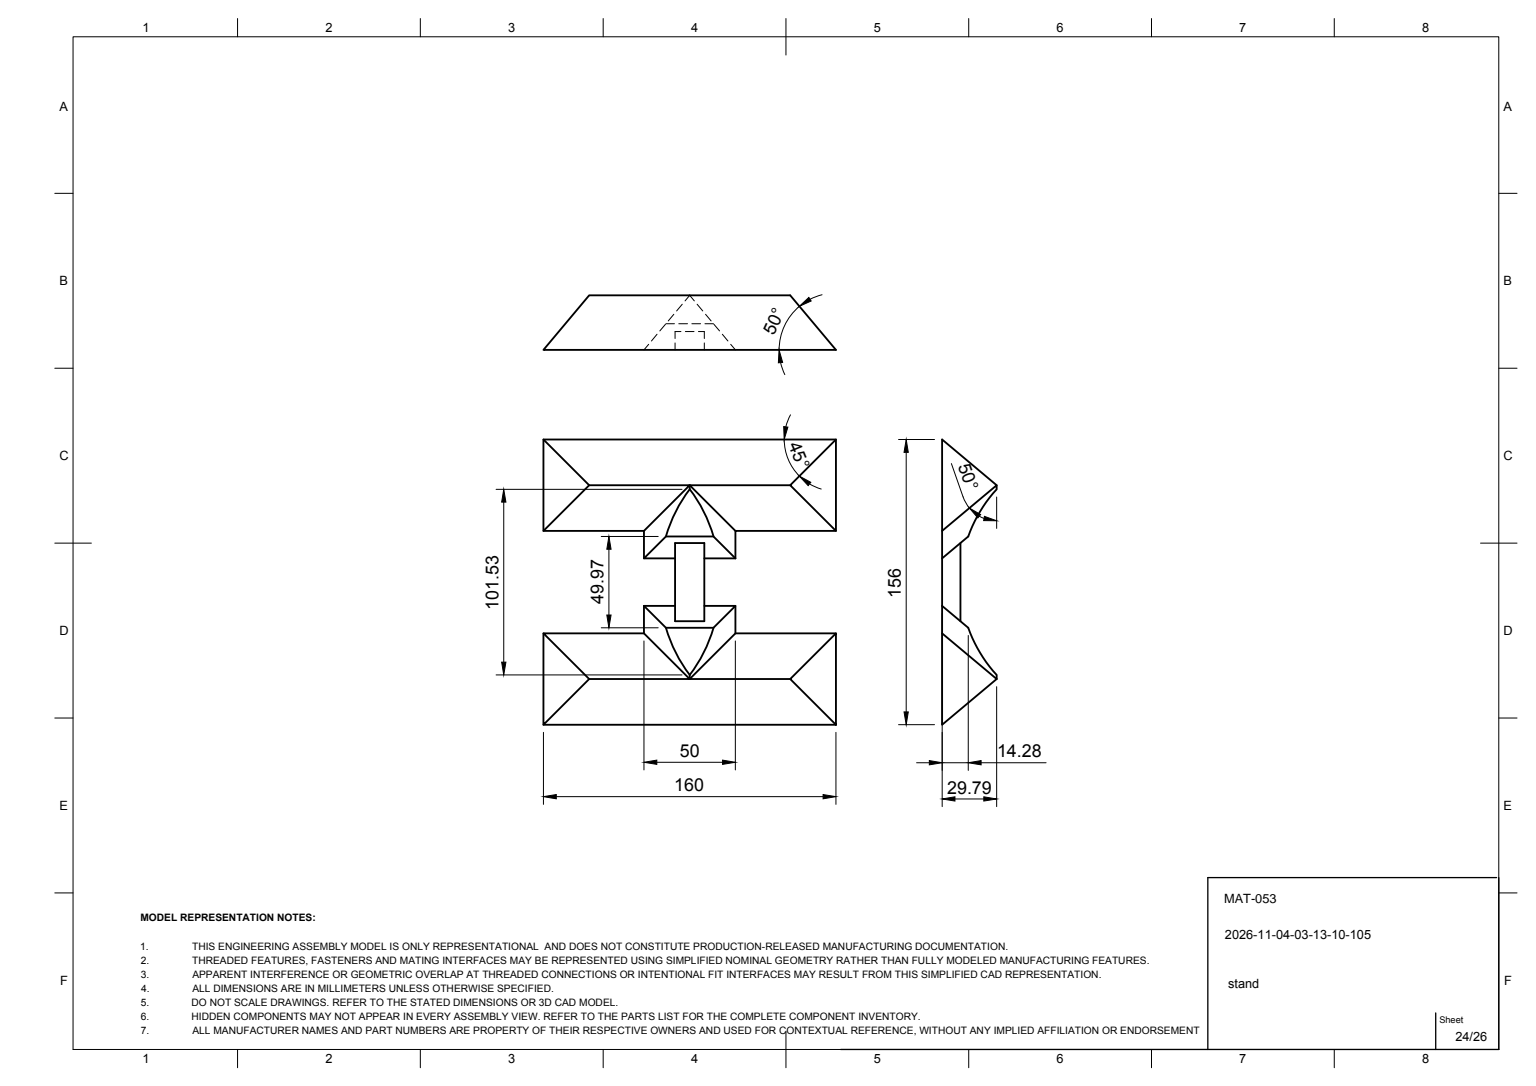
ISO-10303-21;
HEADER;
FILE_DESCRIPTION (('STEP AP214'),
    '1' );
FILE_NAME ('stand.step',
    '2026-10-10T03:43:58',
    ( '' ),
    ( '' ),
    'SwSTEP 2.0',
    'SolidWorks 2026',
    '' );
FILE_SCHEMA (( 'AUTOMOTIVE_DESIGN' ));
ENDSEC;

DATA;
#146=EDGE_LOOP ( 'NONE', ( #8104, #20994, #5292, #47649 ) ) ;
#193=( BOUNDED_CURVE ( )  B_SPLINE_CURVE ( 3, ( #51309, #3119, #36157, #51647 ),
 .UNSPECIFIED., .F., .F. ) 
 B_SPLINE_CURVE_WITH_KNOTS ( ( 4, 4 ),
 ( 0.3396391817068888930, 0.7435323497954801075 ),
 .UNSPECIFIED. ) 
 CURVE ( )  GEOMETRIC_REPRESENTATION_ITEM ( )  RATIONAL_B_SPLINE_CURVE ( ( 1.000000000000000000, 0.9864519964717846090, 0.9864519964717846090, 1.000000000000000000 ) ) 
 REPRESENTATION_ITEM ( '' )  );
#273=CARTESIAN_POINT ( 'NONE',  ( -34.39099631177280969, 10.00000000000000000, -33.00000000000000000 ) ) ;
#625=( BOUNDED_CURVE ( )  B_SPLINE_CURVE ( 3, ( #39954, #62719, #29065, #46526 ),
 .UNSPECIFIED., .F., .F. ) 
 B_SPLINE_CURVE_WITH_KNOTS ( ( 4, 4 ),
 ( 3.481231835296680899, 3.885125003385272446 ),
 .UNSPECIFIED. ) 
 CURVE ( )  GEOMETRIC_REPRESENTATION_ITEM ( )  RATIONAL_B_SPLINE_CURVE ( ( 1.000000000000000000, 0.9864519964717846090, 0.9864519964717846090, 1.000000000000000000 ) ) 
 REPRESENTATION_ITEM ( '' )  );
#713=AXIS2_PLACEMENT_3D ( 'NONE', #6914, #44550, #24147 ) ;
#793=DIRECTION ( 'NONE',  ( -1.661094098900087138E-16, 0.6427876096865404731, 0.7660444431189771253 ) ) ;
#1281=CARTESIAN_POINT ( 'NONE',  ( -26.00000000000000000, 0.000000000000000000, -2.818925648462311923E-15 ) ) ;
#1484=DIRECTION ( 'NONE',  ( 0.000000000000000000, -1.000000000000000000, 0.000000000000000000 ) ) ;
#1494=ADVANCED_FACE ( 'NONE', ( #31724 ), #63402, .T. ) ;
#1497=LINE ( 'NONE', #6064, #10599 ) ;
#1562=DIRECTION ( 'NONE',  ( -1.393823445737823288E-16, 0.7660444431189770143, 0.6427876096865403621 ) ) ;
#1581=VECTOR ( 'NONE', #15769, 1000.000000000000000 ) ;
#1761=EDGE_CURVE ( 'NONE', #54242, #40885, #49448, .T. ) ;
#1806=LINE ( 'NONE', #55245, #35511 ) ;
#1841=CARTESIAN_POINT ( 'NONE',  ( -12.99999999999999645, 0.000000000000000000, -33.00000000000000000 ) ) ;
#1965=CARTESIAN_POINT ( 'NONE',  ( 45.69927128652683734, 36.58596684574255420, -74.30072871347310581 ) ) ;
#2144=LINE ( 'NONE', #35537, #4043 ) ;
#2191=ORIENTED_EDGE ( 'NONE', *, *, #45440, .F. ) ;
#2230=ORIENTED_EDGE ( 'NONE', *, *, #34718, .T. ) ;
#2285=DIRECTION ( 'NONE',  ( 0.5407162030609372616, -0.6444004775717706579, -0.5407162030609374836 ) ) ;
#2317=CARTESIAN_POINT ( 'NONE',  ( 14.99999999999997158, 0.000000000000000000, -0.000000000000000000 ) ) ;
#2392=VERTEX_POINT ( 'NONE', #7790 ) ;
#2515=LINE ( 'NONE', #29246, #19698 ) ;
#2527=ADVANCED_FACE ( 'NONE', ( #21112 ), #68930, .T. ) ;
#2596=DIRECTION ( 'NONE',  ( -2.168404344971009361E-16, 0.000000000000000000, 1.000000000000000000 ) ) ;
#2611=PLANE ( 'NONE',  #12739 ) ;
#2686=FACE_OUTER_BOUND ( 'NONE', #48013, .T. ) ;
#2724=ORIENTED_EDGE ( 'NONE', *, *, #21371, .T. ) ;
#2912=VERTEX_POINT ( 'NONE', #20576 ) ;
#3017=ORIENTED_EDGE ( 'NONE', *, *, #44711, .T. ) ;
#3061=ORIENTED_EDGE ( 'NONE', *, *, #6840, .F. ) ;
#3119=CARTESIAN_POINT ( 'NONE',  ( 21.57182537987934978, 17.67134260003773960, -35.17198294190094288 ) ) ;
#3171=EDGE_LOOP ( 'NONE', ( #50531, #3061, #20090 ) ) ;
#3185=DIRECTION ( 'NONE',  ( -2.168404344971009361E-16, 0.000000000000000000, 1.000000000000000000 ) ) ;
#3231=CARTESIAN_POINT ( 'NONE',  ( 14.99999999999997158, 0.000000000000000000, -50.00000000000000000 ) ) ;
#3532=APPLICATION_CONTEXT ( 'automotive_design' ) ;
#3575=EDGE_LOOP ( 'NONE', ( #20280, #65714, #25182, #9840, #14109 ) ) ;
#3588=PRODUCT_DEFINITION_SHAPE ( 'NONE', 'NONE',  #45241 ) ;
#3605=DIRECTION ( 'NONE',  ( -0.000000000000000000, -0.000000000000000000, 1.000000000000000000 ) ) ;
#3821=ADVANCED_FACE ( 'NONE', ( #39549 ), #2611, .T. ) ;
#3956=LINE ( 'NONE', #25073, #49414 ) ;
#3992=CARTESIAN_POINT ( 'NONE',  ( 0.000000000000000000, 0.000000000000000000, -50.00000000000000000 ) ) ;
#4002=LINE ( 'NONE', #9970, #39539 ) ;
#4043=VECTOR ( 'NONE', #45035, 1000.000000000000000 ) ;
#4119=LINE ( 'NONE', #41409, #61177 ) ;
#4213=DIRECTION ( 'NONE',  ( 1.000000000000000000, -0.000000000000000000, 0.000000000000000000 ) ) ;
#4408=LINE ( 'NONE', #25872, #23224 ) ;
#4594=ADVANCED_FACE ( 'NONE', ( #49482 ), #33688, .F. ) ;
#4687=CARTESIAN_POINT ( 'NONE',  ( 8.390996311772815019, 10.00000000000000000, -33.00000000000000000 ) ) ;
#4737=EDGE_LOOP ( 'NONE', ( #2724, #13378, #43528, #13191 ) ) ;
#4784=DIRECTION ( 'NONE',  ( 8.673617379884039170E-17, 1.033681467326434846E-16, 1.000000000000000000 ) ) ;
#4834=VECTOR ( 'NONE', #51632, 1000.000000000000000 ) ;
#4901=DIRECTION ( 'NONE',  ( 0.6427876096865403621, -0.7660444431189770143, 1.393823445737823288E-16 ) ) ;
#4994=VERTEX_POINT ( 'NONE', #18285 ) ;
#5189=ORIENTED_EDGE ( 'NONE', *, *, #28493, .T. ) ;
#5193=EDGE_CURVE ( 'NONE', #30932, #4994, #40774, .T. ) ;
#5249=FACE_OUTER_BOUND ( 'NONE', #17680, .T. ) ;
#5292=ORIENTED_EDGE ( 'NONE', *, *, #45012, .T. ) ;
#5325=EDGE_CURVE ( 'NONE', #62792, #66752, #31273, .T. ) ;
#5335=DIRECTION ( 'NONE',  ( -0.7660444431189771253, 0.6427876096865404731, 0.000000000000000000 ) ) ;
#5465=VERTEX_POINT ( 'NONE', #273 ) ;
#5614=EDGE_LOOP ( 'NONE', ( #66785, #60378, #47106, #7908 ) ) ;
#5643=CARTESIAN_POINT ( 'NONE',  ( 37.76691715686636996, 29.79383981485516841, -24.99999999999999645 ) ) ;
#5828=PLANE ( 'NONE',  #42178 ) ;
#5906=EDGE_CURVE ( 'NONE', #52737, #43093, #57568, .T. ) ;
#6064=CARTESIAN_POINT ( 'NONE',  ( 11.98601804829806383, 14.28438006995820508, 82.99999999999998579 ) ) ;
#6095=ADVANCED_FACE ( 'NONE', ( #31440 ), #33082, .T. ) ;
#6395=ORIENTED_EDGE ( 'NONE', *, *, #53817, .T. ) ;
#6399=AXIS2_PLACEMENT_3D ( 'NONE', #58013, #42520, #46760 ) ;
#6403=ORIENTED_EDGE ( 'NONE', *, *, #61855, .T. ) ;
#6489=ORIENTED_EDGE ( 'NONE', *, *, #62229, .T. ) ;
#6521=CARTESIAN_POINT ( 'NONE',  ( -37.98601804829807094, 14.28438006995821219, -38.01398195170192906 ) ) ;
#6640=FILL_AREA_STYLE_COLOUR ( '', #26224 ) ;
#6752=LINE ( 'NONE', #54222, #44139 ) ;
#6808=EDGE_CURVE ( 'NONE', #52737, #49963, #59288, .T. ) ;
#6840=EDGE_CURVE ( 'NONE', #10412, #60955, #55768, .T. ) ;
#6914=CARTESIAN_POINT ( 'NONE',  ( -25.99999999999994671, 0.000000000000000000, -104.9999999999999858 ) ) ;
#7029=ORIENTED_EDGE ( 'NONE', *, *, #45012, .F. ) ;
#7036=EDGE_LOOP ( 'NONE', ( #18856, #65533, #68042 ) ) ;
#7077=ORIENTED_EDGE ( 'NONE', *, *, #12957, .F. ) ;
#7275=PLANE ( 'NONE',  #36813 ) ;
#7545=DIRECTION ( 'NONE',  ( -1.000000000000000000, 0.000000000000000000, -0.000000000000000000 ) ) ;
#7708=VERTEX_POINT ( 'NONE', #8980 ) ;
#7790=CARTESIAN_POINT ( 'NONE',  ( -25.99999999999998934, 0.000000000000000000, -50.00000000000000000 ) ) ;
#7908=ORIENTED_EDGE ( 'NONE', *, *, #5906, .F. ) ;
#7927=ORIENTED_EDGE ( 'NONE', *, *, #36685, .T. ) ;
#7960=FACE_OUTER_BOUND ( 'NONE', #31655, .T. ) ;
#8104=ORIENTED_EDGE ( 'NONE', *, *, #5325, .F. ) ;
#8310=CARTESIAN_POINT ( 'NONE',  ( 48.91942932610495376, 19.16407787157945108, 38.91942932610497508 ) ) ;
#8319=DIRECTION ( 'NONE',  ( 1.000000000000000000, 0.000000000000000000, 0.000000000000000000 ) ) ;
#8444=CYLINDRICAL_SURFACE ( 'NONE', #53975, 75.00000000000001421 ) ;
#8520=VERTEX_POINT ( 'NONE', #36152 ) ;
#8591=EDGE_CURVE ( 'NONE', #52737, #53508, #16066, .T. ) ;
#8980=CARTESIAN_POINT ( 'NONE',  ( 11.98601804829806561, 14.28438006995821219, -38.01398195170192906 ) ) ;
#9083=LINE ( 'NONE', #68181, #56913 ) ;
#9198=CARTESIAN_POINT ( 'NONE',  ( -25.99999999999998934, 0.000000000000000000, -50.00000000000000000 ) ) ;
#9199=CARTESIAN_POINT ( 'NONE',  ( -40.99999999999994316, 0.000000000000000000, -104.9999999999999858 ) ) ;
#9378=CARTESIAN_POINT ( 'NONE',  ( -65.99999999999997158, 29.79383981485517197, -2.367957528293540247E-14 ) ) ;
#9391=ADVANCED_FACE ( 'NONE', ( #10501 ), #15452, .T. ) ;
#9660=CARTESIAN_POINT ( 'NONE',  ( -36.61438981621041933, -5.226566692248928447, -54.38561018378954515 ) ) ;
#9758=LINE ( 'NONE', #15026, #4834 ) ;
#9840=ORIENTED_EDGE ( 'NONE', *, *, #30834, .F. ) ;
#9859=VECTOR ( 'NONE', #53368, 1000.000000000000000 ) ;
#9970=CARTESIAN_POINT ( 'NONE',  ( 0.000000000000000000, 0.000000000000000000, -33.00000000000000000 ) ) ;
#9978=CARTESIAN_POINT ( 'NONE',  ( 0.000000000000000000, 0.000000000000000000, -33.00000000000000000 ) ) ;
#10324=CARTESIAN_POINT ( 'NONE',  ( -3.469446951953614189E-15, 0.000000000000000000, -17.00000000000000355 ) ) ;
#10345=EDGE_LOOP ( 'NONE', ( #24574, #33856, #6403 ) ) ;
#10412=VERTEX_POINT ( 'NONE', #57416 ) ;
#10439=ORIENTED_EDGE ( 'NONE', *, *, #58459, .T. ) ;
#10501=FACE_OUTER_BOUND ( 'NONE', #5614, .T. ) ;
#10587=VECTOR ( 'NONE', #12206, 1000.000000000000114 ) ;
#10599=VECTOR ( 'NONE', #44406, 1000.000000000000000 ) ;
#10755=ORIENTED_EDGE ( 'NONE', *, *, #61855, .F. ) ;
#10830=DIRECTION ( 'NONE',  ( 0.000000000000000000, 0.000000000000000000, -1.000000000000000000 ) ) ;
#10864=CARTESIAN_POINT ( 'NONE',  ( -26.00000000000000000, 0.000000000000000000, -2.818925648462311923E-15 ) ) ;
#10931=DIRECTION ( 'NONE',  ( -2.724194322196142817E-16, 0.6427876096865404731, 0.7660444431189771253 ) ) ;
#11112=FACE_OUTER_BOUND ( 'NONE', #3171, .T. ) ;
#11205=LINE ( 'NONE', #31985, #66301 ) ;
#11331=CARTESIAN_POINT ( 'NONE',  ( -37.98601804829808515, 14.28438006995824772, -11.98601804829809581 ) ) ;
#11336=LINE ( 'NONE', #54236, #62534 ) ;
#11370=CARTESIAN_POINT ( 'NONE',  ( -12.99999999999999822, 10.00000000000000000, -17.00000000000000355 ) ) ;
#11437=CARTESIAN_POINT ( 'NONE',  ( -65.99999999999998579, 29.79383981485516841, -1.674068137902818041E-14 ) ) ;
#11515=LINE ( 'NONE', #9198, #39329 ) ;
#11760=CARTESIAN_POINT ( 'NONE',  ( -25.99999999999998934, 0.000000000000000000, -50.00000000000000000 ) ) ;
#11826=DIRECTION ( 'NONE',  ( 0.5407162030609375947, -0.6444004775717707689, -0.5407162030609372616 ) ) ;
#12206=DIRECTION ( 'NONE',  ( -0.6427876096865403621, 0.7660444431189770143, -5.360859406683936151E-17 ) ) ;
#12293=ORIENTED_EDGE ( 'NONE', *, *, #16445, .T. ) ;
#12294=ORIENTED_EDGE ( 'NONE', *, *, #61559, .T. ) ;
#12424=CARTESIAN_POINT ( 'NONE',  ( 7.632783294297949638E-15, 0.000000000000000000, 55.00000000000001421 ) ) ;
#12567=ORIENTED_EDGE ( 'NONE', *, *, #34694, .T. ) ;
#12724=VECTOR ( 'NONE', #21195, 1000.000000000000114 ) ;
#12739=AXIS2_PLACEMENT_3D ( 'NONE', #11760, #33932, #1562 ) ;
#12957=EDGE_CURVE ( 'NONE', #34803, #30932, #56987, .T. ) ;
#12975=ORIENTED_EDGE ( 'NONE', *, *, #17452, .F. ) ;
#13191=ORIENTED_EDGE ( 'NONE', *, *, #47317, .F. ) ;
#13222=VECTOR ( 'NONE', #28910, 1000.000000000000114 ) ;
#13378=ORIENTED_EDGE ( 'NONE', *, *, #37390, .T. ) ;
#13701=CARTESIAN_POINT ( 'NONE',  ( 14.99999999999998579, 0.000000000000000000, -0.000000000000000000 ) ) ;
#13768=EDGE_CURVE ( 'NONE', #40885, #66752, #11205, .T. ) ;
#13823=EDGE_CURVE ( 'NONE', #41104, #30932, #38646, .T. ) ;
#14076=EDGE_CURVE ( 'NONE', #43093, #19218, #48063, .T. ) ;
#14109=ORIENTED_EDGE ( 'NONE', *, *, #1761, .F. ) ;
#14148=ORIENTED_EDGE ( 'NONE', *, *, #42769, .F. ) ;
#14190=ORIENTED_EDGE ( 'NONE', *, *, #62229, .F. ) ;
#14248=LINE ( 'NONE', #9660, #66765 ) ;
#14517=ORIENTED_EDGE ( 'NONE', *, *, #45734, .F. ) ;
#14520=DIRECTION ( 'NONE',  ( -0.5407162030609372616, -0.6444004775717706579, -0.5407162030609377057 ) ) ;
#14586=AXIS2_PLACEMENT_3D ( 'NONE', #63739, #5335, #54186 ) ;
#14782=VERTEX_POINT ( 'NONE', #54826 ) ;
#15026=CARTESIAN_POINT ( 'NONE',  ( -2.914335439641035288E-14, 0.000000000000000000, -104.9999999999999858 ) ) ;
#15262=DIRECTION ( 'NONE',  ( 0.5407162030609374836, -0.6444004775717707689, -0.5407162030609372616 ) ) ;
#15452=PLANE ( 'NONE',  #6399 ) ;
#15769=DIRECTION ( 'NONE',  ( -1.000000000000000000, -0.000000000000000000, -1.334402673828313339E-16 ) ) ;
#15945=AXIS2_PLACEMENT_3D ( 'NONE', #21071, #16124, #68228 ) ;
#16017=ORIENTED_EDGE ( 'NONE', *, *, #45734, .T. ) ;
#16066=LINE ( 'NONE', #47722, #55764 ) ;
#16124=DIRECTION ( 'NONE',  ( 0.000000000000000000, 0.6427876096865404731, 0.7660444431189771253 ) ) ;
#16217=ORIENTED_EDGE ( 'NONE', *, *, #13823, .F. ) ;
#16269=FACE_OUTER_BOUND ( 'NONE', #3575, .T. ) ;
#16321=ORIENTED_EDGE ( 'NONE', *, *, #13768, .F. ) ;
#16374=CARTESIAN_POINT ( 'NONE',  ( -63.76691715686636996, 29.79383981485516841, -25.00000000000000711 ) ) ;
#16445=EDGE_CURVE ( 'NONE', #43093, #41688, #53164, .T. ) ;
#16499=SURFACE_STYLE_USAGE ( .BOTH. , #17898 ) ;
#16560=DIRECTION ( 'NONE',  ( -1.393823445737823288E-16, -0.7660444431189770143, 0.6427876096865403621 ) ) ;
#16724=DIRECTION ( 'NONE',  ( -3.035766082959413401E-16, 1.033681467326434846E-16, 1.000000000000000000 ) ) ;
#16895=VERTEX_POINT ( 'NONE', #50258 ) ;
#16934=EDGE_LOOP ( 'NONE', ( #44814, #6395, #30494, #3017 ) ) ;
#16951=ORIENTED_EDGE ( 'NONE', *, *, #55915, .T. ) ;
#17175=CARTESIAN_POINT ( 'NONE',  ( 14.99999999999997158, 0.000000000000000000, 0.000000000000000000 ) ) ;
#17310=PLANE ( 'NONE',  #63872 ) ;
#17381=( NAMED_UNIT ( * ) SI_UNIT ( $, .STERADIAN. ) SOLID_ANGLE_UNIT ( ) );
#17452=EDGE_CURVE ( 'NONE', #5465, #2912, #28994, .T. ) ;
#17680=EDGE_LOOP ( 'NONE', ( #14190, #12567, #57398, #24199, #58595, #12975, #31349, #24377 ) ) ;
#17898=SURFACE_SIDE_STYLE ('',( #54818 ) ) ;
#18285=CARTESIAN_POINT ( 'NONE',  ( 14.99999999999998579, 0.000000000000000000, 55.00000000000001421 ) ) ;
#18391=( GEOMETRIC_REPRESENTATION_CONTEXT ( 3 ) GLOBAL_UNCERTAINTY_ASSIGNED_CONTEXT ( ( #24754 ) ) GLOBAL_UNIT_ASSIGNED_CONTEXT ( ( #33734, #65747, #48828 ) ) REPRESENTATION_CONTEXT ( 'NONE', 'WORKASPACE' ) );
#18429=UNCERTAINTY_MEASURE_WITH_UNIT (LENGTH_MEASURE( 1.000000000000000082E-05 ), #44825, 'distance_accuracy_value', 'NONE');
#18486=DIRECTION ( 'NONE',  ( 0.000000000000000000, 0.000000000000000000, 1.000000000000000000 ) ) ;
#18712=CARTESIAN_POINT ( 'NONE',  ( 0.000000000000000000, 10.00000000000000000, 0.000000000000000000 ) ) ;
#18856=ORIENTED_EDGE ( 'NONE', *, *, #55915, .F. ) ;
#19187=EDGE_LOOP ( 'NONE', ( #32911, #47972, #5189, #24006, #39056 ) ) ;
#19218=VERTEX_POINT ( 'NONE', #9199 ) ;
#19287=DIRECTION ( 'NONE',  ( 1.734723475976807094E-16, 0.000000000000000000, 1.000000000000000000 ) ) ;
#19348=VECTOR ( 'NONE', #47084, 999.9999999999998863 ) ;
#19421=DIRECTION ( 'NONE',  ( 1.063100223296055310E-16, 0.6427876096865404731, 0.7660444431189771253 ) ) ;
#19431=CARTESIAN_POINT ( 'NONE',  ( -37.98601804829807094, 14.28438006995819798, 82.99999999999997158 ) ) ;
#19505=LINE ( 'NONE', #50138, #36823 ) ;
#19529=EDGE_LOOP ( 'NONE', ( #25599, #61255, #48711, #10755 ) ) ;
#19570=CARTESIAN_POINT ( 'NONE',  ( 14.99999999999998579, 0.000000000000000000, 0.000000000000000000 ) ) ;
#19637=VERTEX_POINT ( 'NONE', #23055 ) ;
#19698=VECTOR ( 'NONE', #24671, 1000.000000000000000 ) ;
#19824=FACE_OUTER_BOUND ( 'NONE', #19979, .T. ) ;
#19856=VECTOR ( 'NONE', #2285, 1000.000000000000114 ) ;
#19979=EDGE_LOOP ( 'NONE', ( #49154, #40536, #24862, #22436, #52944 ) ) ;
#19981=VERTEX_POINT ( 'NONE', #5643 ) ;
#20090=ORIENTED_EDGE ( 'NONE', *, *, #61247, .T. ) ;
#20129=DIRECTION ( 'NONE',  ( -1.000000000000000000, 0.000000000000000000, 1.387778780781445182E-16 ) ) ;
#20242=ORIENTED_EDGE ( 'NONE', *, *, #49797, .T. ) ;
#20280=ORIENTED_EDGE ( 'NONE', *, *, #37541, .F. ) ;
#20576=CARTESIAN_POINT ( 'NONE',  ( -34.39099631177280969, 10.00000000000000000, -17.00000000000000711 ) ) ;
#20754=CARTESIAN_POINT ( 'NONE',  ( 64.99999999999998579, 0.000000000000000000, -1.127570259384924454E-14 ) ) ;
#20994=ORIENTED_EDGE ( 'NONE', *, *, #62728, .T. ) ;
#21071=CARTESIAN_POINT ( 'NONE',  ( 0.000000000000000000, 0.000000000000000000, 0.000000000000000000 ) ) ;
#21112=FACE_OUTER_BOUND ( 'NONE', #19187, .T. ) ;
#21170=CARTESIAN_POINT ( 'NONE',  ( 0.000000000000000000, 0.000000000000000000, 0.000000000000000000 ) ) ;
#21192=EDGE_CURVE ( 'NONE', #27437, #60955, #9758, .T. ) ;
#21195=DIRECTION ( 'NONE',  ( -0.5407162030609373726, -0.6444004775717707689, 0.5407162030609373726 ) ) ;
#21247=DIRECTION ( 'NONE',  ( -1.000000000000000000, -0.000000000000000000, -1.334402673828313339E-16 ) ) ;
#21371=EDGE_CURVE ( 'NONE', #5465, #65127, #37510, .T. ) ;
#21416=DIRECTION ( 'NONE',  ( -2.168404344971009361E-16, 0.000000000000000000, 1.000000000000000000 ) ) ;
#21569=ADVANCED_FACE ( 'NONE', ( #23086 ), #61406, .F. ) ;
#21623=PLANE ( 'NONE',  #41096 ) ;
#21762=DIRECTION ( 'NONE',  ( 2.168404344971009361E-16, 0.000000000000000000, -1.000000000000000000 ) ) ;
#21859=ORIENTED_EDGE ( 'NONE', *, *, #34694, .F. ) ;
#21873=PRODUCT_DEFINITION_CONTEXT ( 'detailed design', #29618, 'design' ) ;
#22053=DIRECTION ( 'NONE',  ( 0.7660444431189771253, 0.6427876096865404731, -1.328875279120069661E-16 ) ) ;
#22140=DIRECTION ( 'NONE',  ( -0.7660444431189771253, 0.6427876096865404731, 0.000000000000000000 ) ) ;
#22247=CARTESIAN_POINT ( 'NONE',  ( -47.57182537987932847, 17.67134260003773605, -14.82801705809906068 ) ) ;
#22365=DIRECTION ( 'NONE',  ( 0.000000000000000000, 0.7660444431189770143, 0.6427876096865403621 ) ) ;
#22436=ORIENTED_EDGE ( 'NONE', *, *, #64725, .T. ) ;
#22651=ORIENTED_EDGE ( 'NONE', *, *, #45440, .T. ) ;
#22841=FACE_OUTER_BOUND ( 'NONE', #38364, .T. ) ;
#22962=ORIENTED_EDGE ( 'NONE', *, *, #40789, .T. ) ;
#23055=CARTESIAN_POINT ( 'NONE',  ( -37.98601804829807094, 14.28438006995821219, -38.01398195170192906 ) ) ;
#23070=LINE ( 'NONE', #2317, #47788 ) ;
#23086=FACE_OUTER_BOUND ( 'NONE', #64231, .T. ) ;
#23224=VECTOR ( 'NONE', #44369, 1000.000000000000000 ) ;
#23322=ORIENTED_EDGE ( 'NONE', *, *, #40841, .T. ) ;
#23370=ORIENTED_EDGE ( 'NONE', *, *, #8591, .F. ) ;
#24006=ORIENTED_EDGE ( 'NONE', *, *, #40841, .F. ) ;
#24007=ORIENTED_EDGE ( 'NONE', *, *, #37141, .F. ) ;
#24147=DIRECTION ( 'NONE',  ( -1.393823445737823288E-16, 0.7660444431189770143, 0.6427876096865403621 ) ) ;
#24150=DIRECTION ( 'NONE',  ( 0.6427876096865403621, -0.7660444431189770143, 1.393823445737823288E-16 ) ) ;
#24199=ORIENTED_EDGE ( 'NONE', *, *, #13768, .T. ) ;
#24244=LINE ( 'NONE', #34793, #29691 ) ;
#24377=ORIENTED_EDGE ( 'NONE', *, *, #28757, .T. ) ;
#24499=DIRECTION ( 'NONE',  ( 0.5407162030609374836, -0.6444004775717707689, 0.5407162030609373726 ) ) ;
#24566=CARTESIAN_POINT ( 'NONE',  ( 0.000000000000000000, 0.000000000000000000, -50.00000000000000000 ) ) ;
#24574=ORIENTED_EDGE ( 'NONE', *, *, #34718, .F. ) ;
#24671=DIRECTION ( 'NONE',  ( -0.5407162030609375947, -0.6444004775717706579, 0.5407162030609372616 ) ) ;
#24743=VECTOR ( 'NONE', #3605, 1000.000000000000000 ) ;
#24754=UNCERTAINTY_MEASURE_WITH_UNIT (LENGTH_MEASURE( 1.000000000000000082E-05 ), #33734, 'distance_accuracy_value', 'NONE');
#24862=ORIENTED_EDGE ( 'NONE', *, *, #30027, .F. ) ;
#25073=CARTESIAN_POINT ( 'NONE',  ( 7.632783294297949638E-15, 0.000000000000000000, 55.00000000000001421 ) ) ;
#25182=ORIENTED_EDGE ( 'NONE', *, *, #8591, .T. ) ;
#25505=DIRECTION ( 'NONE',  ( 0.5407162030609374836, -0.6444004775717707689, -0.5407162030609372616 ) ) ;
#25589=VECTOR ( 'NONE', #57751, 1000.000000000000000 ) ;
#25599=ORIENTED_EDGE ( 'NONE', *, *, #56469, .F. ) ;
#25809=DIRECTION ( 'NONE',  ( -0.6427876096865403621, -0.7660444431189770143, 0.000000000000000000 ) ) ;
#25828=CARTESIAN_POINT ( 'NONE',  ( -40.61870061263184084, 17.42188897416313154, -35.38129938736816626 ) ) ;
#25872=CARTESIAN_POINT ( 'NONE',  ( -26.00000000000000000, 0.000000000000000000, -2.818925648462311923E-15 ) ) ;
#26086=FACE_OUTER_BOUND ( 'NONE', #62478, .T. ) ;
#26224=COLOUR_RGB ( '',0.7921568627450980005, 0.8196078431372548767, 0.9333333333333333481 ) ;
#26319=LINE ( 'NONE', #58312, #9859 ) ;
#26347=PLANE ( 'NONE',  #15945 ) ;
#26538=VERTEX_POINT ( 'NONE', #36286 ) ;
#26772=ORIENTED_EDGE ( 'NONE', *, *, #59613, .F. ) ;
#26870=LINE ( 'NONE', #11370, #32136 ) ;
#27104=( BOUNDED_CURVE ( )  B_SPLINE_CURVE ( 3, ( #16374, #43440, #27263, #6521 ),
 .UNSPECIFIED., .F., .F. ) 
 B_SPLINE_CURVE_WITH_KNOTS ( ( 4, 4 ),
 ( 5.539652957384106458, 5.943546125472697561 ),
 .UNSPECIFIED. ) 
 CURVE ( )  GEOMETRIC_REPRESENTATION_ITEM ( )  RATIONAL_B_SPLINE_CURVE ( ( 1.000000000000000000, 0.9864519964717846090, 0.9864519964717846090, 1.000000000000000000 ) ) 
 REPRESENTATION_ITEM ( '' )  );
#27164=CARTESIAN_POINT ( 'NONE',  ( -63.76691715686636996, 29.79383981485516841, -25.00000000000000711 ) ) ;
#27198=ORIENTED_EDGE ( 'NONE', *, *, #12957, .T. ) ;
#27246=CARTESIAN_POINT ( 'NONE',  ( 11.98601804829804607, 14.28438006995819443, -11.98601804829804607 ) ) ;
#27263=CARTESIAN_POINT ( 'NONE',  ( -47.57182537987935689, 17.67134260003773960, -35.17198294190094288 ) ) ;
#27284=CARTESIAN_POINT ( 'NONE',  ( -2.914335439641035288E-14, 0.000000000000000000, -104.9999999999999858 ) ) ;
#27408=DIRECTION ( 'NONE',  ( -0.6427876096865403621, -0.7660444431189770143, 0.000000000000000000 ) ) ;
#27412=ORIENTED_EDGE ( 'NONE', *, *, #58454, .T. ) ;
#27437=VERTEX_POINT ( 'NONE', #62716 ) ;
#27459=ORIENTED_EDGE ( 'NONE', *, *, #66369, .T. ) ;
#27596=DIRECTION ( 'NONE',  ( 1.000000000000000000, 0.000000000000000000, 4.943961906533900219E-16 ) ) ;
#27741=PRESENTATION_STYLE_ASSIGNMENT (( #16499 ) ) ;
#28104=CARTESIAN_POINT ( 'NONE',  ( -91.00000000000001421, 0.000000000000000000, 54.99999999999999289 ) ) ;
#28298=CLOSED_SHELL ( 'NONE', ( #29139, #35185, #44463, #1494, #48003, #66986, #34800, #51237, #2527, #4594, #60335, #34825, #37773, #28588, #9391, #3821, #49058, #47702, #33911, #6095, #21569, #66800 ) ) ;
#28493=EDGE_CURVE ( 'NONE', #42670, #62968, #38570, .T. ) ;
#28588=ADVANCED_FACE ( 'NONE', ( #7960 ), #40651, .T. ) ;
#28757=EDGE_CURVE ( 'NONE', #8520, #2392, #4408, .T. ) ;
#28839=VECTOR ( 'NONE', #21416, 1000.000000000000000 ) ;
#28910=DIRECTION ( 'NONE',  ( 0.6427876096865403621, -0.7660444431189770143, 1.393823445737823288E-16 ) ) ;
#28994=LINE ( 'NONE', #46534, #33877 ) ;
#29065=CARTESIAN_POINT ( 'NONE',  ( 30.28348399776037070, 22.91216519805201202, -19.22558936715840261 ) ) ;
#29139=ADVANCED_FACE ( 'NONE', ( #22841 ), #44282, .T. ) ;
#29201=AXIS2_PLACEMENT_3D ( 'NONE', #10864, #31306, #4901 ) ;
#29246=CARTESIAN_POINT ( 'NONE',  ( -74.91942932610496086, 19.16407787157945108, 38.91942932610496086 ) ) ;
#29279=LINE ( 'NONE', #35247, #49292 ) ;
#29618=APPLICATION_CONTEXT ( 'automotive_design' ) ;
#29691=VECTOR ( 'NONE', #19287, 1000.000000000000000 ) ;
#30027=EDGE_CURVE ( 'NONE', #41104, #19981, #48414, .T. ) ;
#30121=CARTESIAN_POINT ( 'NONE',  ( -40.99999999999997868, 0.000000000000000000, -6.071532165918823253E-15 ) ) ;
#30311=AXIS2_PLACEMENT_3D ( 'NONE', #47516, #10931, #16560 ) ;
#30494=ORIENTED_EDGE ( 'NONE', *, *, #6840, .T. ) ;
#30563=PRODUCT ( 'stand', 'stand', '', ( #31176 ) ) ;
#30656=VECTOR ( 'NONE', #64953, 1000.000000000000000 ) ;
#30703=CARTESIAN_POINT ( 'NONE',  ( -60.30072871347308450, 36.58596684574257552, -74.30072871347313423 ) ) ;
#30720=AXIS2_PLACEMENT_3D ( 'NONE', #17175, #54454, #58445 ) ;
#30834=EDGE_CURVE ( 'NONE', #40885, #53508, #26319, .T. ) ;
#30876=CARTESIAN_POINT ( 'NONE',  ( -65.99999999999995737, 29.79383981485516131, -25.00000000000001066 ) ) ;
#30915=( GEOMETRIC_REPRESENTATION_CONTEXT ( 3 ) GLOBAL_UNCERTAINTY_ASSIGNED_CONTEXT ( ( #18429 ) ) GLOBAL_UNIT_ASSIGNED_CONTEXT ( ( #44825, #44472, #17381 ) ) REPRESENTATION_CONTEXT ( 'NONE', 'WORKASPACE' ) );
#30919=VECTOR ( 'NONE', #16724, 1000.000000000000000 ) ;
#30932=VERTEX_POINT ( 'NONE', #19570 ) ;
#30952=ORIENTED_EDGE ( 'NONE', *, *, #65618, .T. ) ;
#31176=PRODUCT_CONTEXT ( 'NONE', #3532, 'mechanical' ) ;
#31273=LINE ( 'NONE', #52700, #1581 ) ;
#31306=DIRECTION ( 'NONE',  ( 0.7660444431189771253, 0.6427876096865404731, 1.661094098900087138E-16 ) ) ;
#31349=ORIENTED_EDGE ( 'NONE', *, *, #47317, .T. ) ;
#31440=FACE_OUTER_BOUND ( 'NONE', #58349, .T. ) ;
#31655=EDGE_LOOP ( 'NONE', ( #24007, #55696, #56742 ) ) ;
#31694=ORIENTED_EDGE ( 'NONE', *, *, #40789, .F. ) ;
#31724=FACE_OUTER_BOUND ( 'NONE', #16934, .T. ) ;
#31985=CARTESIAN_POINT ( 'NONE',  ( -26.00000000000000000, 0.000000000000000000, -2.818925648462311923E-15 ) ) ;
#32136=VECTOR ( 'NONE', #21247, 1000.000000000000000 ) ;
#32301=VECTOR ( 'NONE', #7545, 1000.000000000000000 ) ;
#32417=PLANE ( 'NONE',  #40441 ) ;
#32614=LINE ( 'NONE', #53706, #10587 ) ;
#32666=ORIENTED_EDGE ( 'NONE', *, *, #5325, .T. ) ;
#32701=VECTOR ( 'NONE', #45076, 1000.000000000000000 ) ;
#32800=CARTESIAN_POINT ( 'NONE',  ( -26.00000000000000000, 0.000000000000000000, -2.818925648462311923E-15 ) ) ;
#32879=EDGE_CURVE ( 'NONE', #7708, #45932, #29279, .T. ) ;
#32911=ORIENTED_EDGE ( 'NONE', *, *, #53817, .F. ) ;
#33082=PLANE ( 'NONE',  #68999 ) ;
#33109=CARTESIAN_POINT ( 'NONE',  ( -12.99999999999999645, 10.00000000000000000, -33.00000000000000000 ) ) ;
#33340=CARTESIAN_POINT ( 'NONE',  ( 0.000000000000000000, 0.000000000000000000, 0.000000000000000000 ) ) ;
#33648=DIRECTION ( 'NONE',  ( -1.000000000000000000, 0.000000000000000000, 0.000000000000000000 ) ) ;
#33653=DIRECTION ( 'NONE',  ( 0.5407162030609372616, -0.6444004775717707689, 0.5407162030609374836 ) ) ;
#33688=PLANE ( 'NONE',  #49827 ) ;
#33734=( LENGTH_UNIT ( ) NAMED_UNIT ( * ) SI_UNIT ( .MILLI., .METRE. ) );
#33856=ORIENTED_EDGE ( 'NONE', *, *, #28493, .F. ) ;
#33877=VECTOR ( 'NONE', #2596, 1000.000000000000000 ) ;
#33911=ADVANCED_FACE ( 'NONE', ( #26086 ), #58094, .T. ) ;
#33932=DIRECTION ( 'NONE',  ( 1.661094098900087138E-16, 0.6427876096865404731, -0.7660444431189771253 ) ) ;
#34345=CARTESIAN_POINT ( 'NONE',  ( -12.99999999999999822, 84.99999999999998579, 82.99999999999998579 ) ) ;
#34438=VECTOR ( 'NONE', #3185, 1000.000000000000000 ) ;
#34694=EDGE_CURVE ( 'NONE', #19637, #54242, #47527, .T. ) ;
#34718=EDGE_CURVE ( 'NONE', #62968, #4994, #3956, .T. ) ;
#34793=CARTESIAN_POINT ( 'NONE',  ( 64.99999999999998579, 0.000000000000000000, -1.127570259384924454E-14 ) ) ;
#34800=ADVANCED_FACE ( 'NONE', ( #38376 ), #42275, .T. ) ;
#34803=VERTEX_POINT ( 'NONE', #21170 ) ;
#34825=ADVANCED_FACE ( 'NONE', ( #59820 ), #32417, .T. ) ;
#35185=ADVANCED_FACE ( 'NONE', ( #5249 ), #53071, .T. ) ;
#35218=MECHANICAL_DESIGN_GEOMETRIC_PRESENTATION_REPRESENTATION('',(#65548),#18391);
#35247=CARTESIAN_POINT ( 'NONE',  ( 14.61870061263185150, 17.42188897416313154, -35.38129938736816626 ) ) ;
#35511=VECTOR ( 'NONE', #65828, 1000.000000000000000 ) ;
#35537=CARTESIAN_POINT ( 'NONE',  ( -25.99999999999999289, 29.79383981485516841, -25.00000000000000000 ) ) ;
#35770=EDGE_LOOP ( 'NONE', ( #27412, #57218, #6489, #30952, #14148 ) ) ;
#35810=ORIENTED_EDGE ( 'NONE', *, *, #61959, .F. ) ;
#36152=CARTESIAN_POINT ( 'NONE',  ( -25.99999999999999289, 0.000000000000000000, -33.00000000000000000 ) ) ;
#36157=CARTESIAN_POINT ( 'NONE',  ( 30.28348399776043465, 22.91216519805204754, -30.77441063284156897 ) ) ;
#36248=DIRECTION ( 'NONE',  ( -0.6427876096865403621, 0.7660444431189770143, 0.000000000000000000 ) ) ;
#36286=CARTESIAN_POINT ( 'NONE',  ( -40.99999999999995737, 0.000000000000000000, -50.00000000000000000 ) ) ;
#36632=DIRECTION ( 'NONE',  ( -1.000000000000000000, 0.000000000000000000, -2.168404344971009361E-16 ) ) ;
#36685=EDGE_CURVE ( 'NONE', #8520, #65221, #40159, .T. ) ;
#36775=VECTOR ( 'NONE', #15262, 1000.000000000000114 ) ;
#36813=AXIS2_PLACEMENT_3D ( 'NONE', #30121, #67405, #24150 ) ;
#36823=VECTOR ( 'NONE', #56805, 1000.000000000000114 ) ;
#36928=ORIENTED_EDGE ( 'NONE', *, *, #37390, .F. ) ;
#37097=VERTEX_POINT ( 'NONE', #27246 ) ;
#37141=EDGE_CURVE ( 'NONE', #41688, #19218, #49037, .T. ) ;
#37151=DIRECTION ( 'NONE',  ( 1.000000000000000000, -0.000000000000000000, 0.000000000000000000 ) ) ;
#37390=EDGE_CURVE ( 'NONE', #65127, #65221, #4002, .T. ) ;
#37510=LINE ( 'NONE', #58963, #30656 ) ;
#37515=CARTESIAN_POINT ( 'NONE',  ( -71.69927128652682313, 36.58596684574255420, -74.30072871347312002 ) ) ;
#37541=EDGE_CURVE ( 'NONE', #37939, #54242, #55901, .T. ) ;
#37726=DIRECTION ( 'NONE',  ( -1.393823445737823288E-16, -0.7660444431189770143, 0.6427876096865403621 ) ) ;
#37773=ADVANCED_FACE ( 'NONE', ( #66568 ), #66916, .F. ) ;
#37939=VERTEX_POINT ( 'NONE', #58739 ) ;
#38290=EDGE_CURVE ( 'NONE', #49963, #14782, #62222, .T. ) ;
#38364=EDGE_LOOP ( 'NONE', ( #31694, #16951, #54456, #50515, #36928, #64829, #47853, #48516 ) ) ;
#38376=FACE_OUTER_BOUND ( 'NONE', #19529, .T. ) ;
#38409=DIRECTION ( 'NONE',  ( -8.673617379884037937E-17, -1.033681467326434969E-16, -1.000000000000000000 ) ) ;
#38570=LINE ( 'NONE', #8310, #52331 ) ;
#38646=LINE ( 'NONE', #60086, #56127 ) ;
#38906=DIRECTION ( 'NONE',  ( -2.126200446592111359E-16, 0.6427876096865404731, -0.7660444431189771253 ) ) ;
#39056=ORIENTED_EDGE ( 'NONE', *, *, #61247, .F. ) ;
#39160=CARTESIAN_POINT ( 'NONE',  ( 65.00000000000000000, 0.000000000000000000, 55.00000000000000711 ) ) ;
#39329=VECTOR ( 'NONE', #36632, 1000.000000000000000 ) ;
#39376=VECTOR ( 'NONE', #39834, 1000.000000000000000 ) ;
#39450=LINE ( 'NONE', #40150, #13222 ) ;
#39539=VECTOR ( 'NONE', #25809, 1000.000000000000114 ) ;
#39549=FACE_OUTER_BOUND ( 'NONE', #35770, .T. ) ;
#39645=ORIENTED_EDGE ( 'NONE', *, *, #5193, .F. ) ;
#39647=AXIS2_PLACEMENT_3D ( 'NONE', #34345, #55788, #33648 ) ;
#39834=DIRECTION ( 'NONE',  ( 0.000000000000000000, 0.000000000000000000, -1.000000000000000000 ) ) ;
#39899=VECTOR ( 'NONE', #49422, 1000.000000000000114 ) ;
#39903=MANIFOLD_SOLID_BREP ( 'Cut-Extrude1', #28298 ) ;
#39954=CARTESIAN_POINT ( 'NONE',  ( 11.98601804829804607, 14.28438006995819443, -11.98601804829804607 ) ) ;
#40118=LINE ( 'NONE', #56636, #34438 ) ;
#40150=CARTESIAN_POINT ( 'NONE',  ( -25.99999999999999289, 0.000000000000000000, -33.00000000000000000 ) ) ;
#40159=LINE ( 'NONE', #1841, #32701 ) ;
#40441=AXIS2_PLACEMENT_3D ( 'NONE', #33109, #53148, #64070 ) ;
#40536=ORIENTED_EDGE ( 'NONE', *, *, #61857, .T. ) ;
#40651=PLANE ( 'NONE',  #713 ) ;
#40676=CARTESIAN_POINT ( 'NONE',  ( 10.61438981621042643, -5.226566692248928447, -54.38561018378954515 ) ) ;
#40774=LINE ( 'NONE', #13701, #63346 ) ;
#40789=EDGE_CURVE ( 'NONE', #37097, #34803, #66126, .T. ) ;
#40841=EDGE_CURVE ( 'NONE', #27437, #62968, #24244, .T. ) ;
#40885=VERTEX_POINT ( 'NONE', #51995 ) ;
#40986=EDGE_CURVE ( 'NONE', #66752, #2912, #32614, .T. ) ;
#41096=AXIS2_PLACEMENT_3D ( 'NONE', #43068, #64893, #64540 ) ;
#41104=VERTEX_POINT ( 'NONE', #66728 ) ;
#41124=CARTESIAN_POINT ( 'NONE',  ( -57.08057067389502492, 19.16407787157944398, 38.91942932610496797 ) ) ;
#41409=CARTESIAN_POINT ( 'NONE',  ( 0.000000000000000000, 0.000000000000000000, -50.00000000000000000 ) ) ;
#41688=VERTEX_POINT ( 'NONE', #61612 ) ;
#41732=DIRECTION ( 'NONE',  ( 3.035766082959412908E-16, -1.033681467326434969E-16, -1.000000000000000000 ) ) ;
#41963=DIRECTION ( 'NONE',  ( 0.000000000000000000, 0.6427876096865404731, -0.7660444431189771253 ) ) ;
#42178=AXIS2_PLACEMENT_3D ( 'NONE', #27284, #38906, #22365 ) ;
#42264=CARTESIAN_POINT ( 'NONE',  ( 8.390996311772823901, 10.00000000000000000, 0.000000000000000000 ) ) ;
#42275=PLANE ( 'NONE',  #14586 ) ;
#42297=LINE ( 'NONE', #58696, #28839 ) ;
#42506=EDGE_CURVE ( 'NONE', #45932, #49158, #4119, .T. ) ;
#42520=DIRECTION ( 'NONE',  ( 0.7660444431189771253, 0.6427876096865404731, 1.661094098900087138E-16 ) ) ;
#42670=VERTEX_POINT ( 'NONE', #56112 ) ;
#42769=EDGE_CURVE ( 'NONE', #52737, #26538, #14248, .T. ) ;
#43024=ORIENTED_EDGE ( 'NONE', *, *, #37141, .T. ) ;
#43068=CARTESIAN_POINT ( 'NONE',  ( -12.99999999999999822, 10.00000000000000000, -17.00000000000000355 ) ) ;
#43093=VERTEX_POINT ( 'NONE', #45293 ) ;
#43440=CARTESIAN_POINT ( 'NONE',  ( -56.28348399776044175, 22.91216519805206531, -30.77441063284156897 ) ) ;
#43528=ORIENTED_EDGE ( 'NONE', *, *, #36685, .F. ) ;
#43565=AXIS2_PLACEMENT_3D ( 'NONE', #3992, #41963, #46896 ) ;
#43857=CARTESIAN_POINT ( 'NONE',  ( 14.99999999999997158, 0.000000000000000000, -104.9999999999999858 ) ) ;
#43928=CARTESIAN_POINT ( 'NONE',  ( 0.000000000000000000, 0.000000000000000000, 0.000000000000000000 ) ) ;
#44117=LINE ( 'NONE', #45527, #19856 ) ;
#44139=VECTOR ( 'NONE', #38409, 1000.000000000000000 ) ;
#44282=PLANE ( 'NONE',  #44551 ) ;
#44369=DIRECTION ( 'NONE',  ( 2.168404344971009361E-16, 0.000000000000000000, -1.000000000000000000 ) ) ;
#44406=DIRECTION ( 'NONE',  ( 0.000000000000000000, 0.000000000000000000, -1.000000000000000000 ) ) ;
#44413=LINE ( 'NONE', #60246, #39376 ) ;
#44463=ADVANCED_FACE ( 'NONE', ( #11112 ), #5828, .T. ) ;
#44472=( NAMED_UNIT ( * ) PLANE_ANGLE_UNIT ( ) SI_UNIT ( $, .RADIAN. ) );
#44550=DIRECTION ( 'NONE',  ( 3.787294545492198744E-16, 0.6427876096865404731, -0.7660444431189771253 ) ) ;
#44551=AXIS2_PLACEMENT_3D ( 'NONE', #43928, #22140, #27408 ) ;
#44558=DIRECTION ( 'NONE',  ( 0.000000000000000000, 0.000000000000000000, 1.000000000000000000 ) ) ;
#44711=EDGE_CURVE ( 'NONE', #60955, #49158, #23070, .T. ) ;
#44814=ORIENTED_EDGE ( 'NONE', *, *, #64725, .F. ) ;
#44822=ORIENTED_EDGE ( 'NONE', *, *, #5906, .T. ) ;
#44825=( LENGTH_UNIT ( ) NAMED_UNIT ( * ) SI_UNIT ( .MILLI., .METRE. ) );
#45012=EDGE_CURVE ( 'NONE', #16895, #2912, #26870, .T. ) ;
#45035=DIRECTION ( 'NONE',  ( 1.000000000000000000, -0.000000000000000000, 2.168404344971009608E-16 ) ) ;
#45076=DIRECTION ( 'NONE',  ( 1.000000000000000000, 0.000000000000000000, 0.000000000000000000 ) ) ;
#45241=PRODUCT_DEFINITION ( 'UNKNOWN', '', #55760, #21873 ) ;
#45256=CARTESIAN_POINT ( 'NONE',  ( -37.98601804829808515, 14.28438006995824772, -11.98601804829809581 ) ) ;
#45293=CARTESIAN_POINT ( 'NONE',  ( -65.99999999999994316, 29.79383981485516486, -80.00000000000000000 ) ) ;
#45376=DIRECTION ( 'NONE',  ( 0.000000000000000000, 0.000000000000000000, -1.000000000000000000 ) ) ;
#45440=EDGE_CURVE ( 'NONE', #41688, #56069, #1806, .T. ) ;
#45527=CARTESIAN_POINT ( 'NONE',  ( 34.30072871347309871, 36.58596684574257552, -74.30072871347312002 ) ) ;
#45734=EDGE_CURVE ( 'NONE', #53508, #14782, #42297, .T. ) ;
#45932=VERTEX_POINT ( 'NONE', #24566 ) ;
#46064=FACE_OUTER_BOUND ( 'NONE', #7036, .T. ) ;
#46190=EDGE_CURVE ( 'NONE', #37097, #19981, #625, .T. ) ;
#46225=LINE ( 'NONE', #25828, #36775 ) ;
#46469=AXIS2_PLACEMENT_3D ( 'NONE', #20754, #22053, #36248 ) ;
#46526=CARTESIAN_POINT ( 'NONE',  ( 37.76691715686636996, 29.79383981485516841, -24.99999999999999645 ) ) ;
#46534=CARTESIAN_POINT ( 'NONE',  ( -34.39099631177282390, 10.00000000000000000, -4.638432934570702075E-15 ) ) ;
#46760=DIRECTION ( 'NONE',  ( 0.6427876096865403621, -0.7660444431189770143, 1.393823445737823288E-16 ) ) ;
#46896=DIRECTION ( 'NONE',  ( 0.000000000000000000, 0.7660444431189770143, 0.6427876096865403621 ) ) ;
#47082=ORIENTED_EDGE ( 'NONE', *, *, #6808, .T. ) ;
#47084=DIRECTION ( 'NONE',  ( 0.5407162030609372616, -0.6444004775717707689, 0.5407162030609375947 ) ) ;
#47101=VECTOR ( 'NONE', #68126, 1000.000000000000114 ) ;
#47106=ORIENTED_EDGE ( 'NONE', *, *, #14076, .F. ) ;
#47228=PLANE ( 'NONE',  #43565 ) ;
#47317=EDGE_CURVE ( 'NONE', #5465, #8520, #39450, .T. ) ;
#47516=CARTESIAN_POINT ( 'NONE',  ( -26.00000000000002132, 0.000000000000000000, 55.00000000000001421 ) ) ;
#47527=LINE ( 'NONE', #19431, #24743 ) ;
#47538=ORIENTED_EDGE ( 'NONE', *, *, #46190, .F. ) ;
#47649=ORIENTED_EDGE ( 'NONE', *, *, #40986, .F. ) ;
#47702=ADVANCED_FACE ( 'NONE', ( #2686 ), #7275, .T. ) ;
#47722=CARTESIAN_POINT ( 'NONE',  ( -36.61438981621043354, -5.226566692248933776, 4.385610183789545147 ) ) ;
#47788=VECTOR ( 'NONE', #18486, 1000.000000000000000 ) ;
#47853=ORIENTED_EDGE ( 'NONE', *, *, #62728, .F. ) ;
#47942=CARTESIAN_POINT ( 'NONE',  ( -90.99999999999998579, 0.000000000000000000, -2.818925648462311528E-14 ) ) ;
#47972=ORIENTED_EDGE ( 'NONE', *, *, #56469, .T. ) ;
#48003=ADVANCED_FACE ( 'NONE', ( #19824 ), #47228, .T. ) ;
#48013=EDGE_LOOP ( 'NONE', ( #47082, #50560, #14517, #23370 ) ) ;
#48063=LINE ( 'NONE', #37515, #58373 ) ;
#48255=SHAPE_REPRESENTATION ( 'stand', ( #66832 ), #30915 ) ;
#48330=FACE_OUTER_BOUND ( 'NONE', #146, .T. ) ;
#48414=LINE ( 'NONE', #48765, #32301 ) ;
#48516=ORIENTED_EDGE ( 'NONE', *, *, #49797, .F. ) ;
#48711=ORIENTED_EDGE ( 'NONE', *, *, #5193, .T. ) ;
#48765=CARTESIAN_POINT ( 'NONE',  ( 0.000000000000000000, 29.79383981485516841, -24.99999999999999645 ) ) ;
#48777=ORIENTED_EDGE ( 'NONE', *, *, #42506, .T. ) ;
#48828=( NAMED_UNIT ( * ) SI_UNIT ( $, .STERADIAN. ) SOLID_ANGLE_UNIT ( ) );
#48957=DIRECTION ( 'NONE',  ( 1.000000000000000000, 0.000000000000000000, 3.556183125752454544E-16 ) ) ;
#49037=LINE ( 'NONE', #65599, #57463 ) ;
#49058=ADVANCED_FACE ( 'NONE', ( #16269 ), #17310, .T. ) ;
#49154=ORIENTED_EDGE ( 'NONE', *, *, #32879, .F. ) ;
#49158=VERTEX_POINT ( 'NONE', #3231 ) ;
#49292=VECTOR ( 'NONE', #66933, 1000.000000000000114 ) ;
#49414=VECTOR ( 'NONE', #20129, 1000.000000000000000 ) ;
#49422=DIRECTION ( 'NONE',  ( -0.5407162030609373726, -0.6444004775717707689, -0.5407162030609372616 ) ) ;
#49448=LINE ( 'NONE', #1281, #53129 ) ;
#49482=FACE_OUTER_BOUND ( 'NONE', #57134, .T. ) ;
#49580=VECTOR ( 'NONE', #14520, 1000.000000000000000 ) ;
#49797=EDGE_CURVE ( 'NONE', #34803, #62792, #65000, .T. ) ;
#49827=AXIS2_PLACEMENT_3D ( 'NONE', #33340, #66053, #59688 ) ;
#49843=CARTESIAN_POINT ( 'NONE',  ( -66.00000000000000000, 29.79383981485516486, 29.99999999999999645 ) ) ;
#49963=VERTEX_POINT ( 'NONE', #49843 ) ;
#50054=PLANE ( 'NONE',  #50697 ) ;
#50138=CARTESIAN_POINT ( 'NONE',  ( 9.372831690575286860E-16, 1.117010584002392767E-15, -17.00000000000000000 ) ) ;
#50258=CARTESIAN_POINT ( 'NONE',  ( 8.390996311772816796, 10.00000000000000000, -17.00000000000000000 ) ) ;
#50409=ORIENTED_EDGE ( 'NONE', *, *, #65618, .F. ) ;
#50515=ORIENTED_EDGE ( 'NONE', *, *, #66369, .F. ) ;
#50530=CARTESIAN_POINT ( 'NONE',  ( 0.000000000000000000, 0.000000000000000000, 0.000000000000000000 ) ) ;
#50531=ORIENTED_EDGE ( 'NONE', *, *, #21192, .T. ) ;
#50560=ORIENTED_EDGE ( 'NONE', *, *, #38290, .T. ) ;
#50564=ORIENTED_EDGE ( 'NONE', *, *, #21192, .F. ) ;
#50697=AXIS2_PLACEMENT_3D ( 'NONE', #12424, #19421, #52799 ) ;
#50824=ADVANCED_BREP_SHAPE_REPRESENTATION ( '', ( #39903, #66832 ), #30915 ) ;
#51007=CARTESIAN_POINT ( 'NONE',  ( -12.99999999999999822, 84.99999999999998579, 82.99999999999998579 ) ) ;
#51054=VECTOR ( 'NONE', #41732, 1000.000000000000000 ) ;
#51237=ADVANCED_FACE ( 'NONE', ( #60604 ), #50054, .T. ) ;
#51309=CARTESIAN_POINT ( 'NONE',  ( 11.98601804829806561, 14.28438006995821219, -38.01398195170192906 ) ) ;
#51632=DIRECTION ( 'NONE',  ( -1.000000000000000000, 0.000000000000000000, 2.775557561562891351E-16 ) ) ;
#51647=CARTESIAN_POINT ( 'NONE',  ( 37.76691715686636996, 29.79383981485516841, -24.99999999999999645 ) ) ;
#51781=LINE ( 'NONE', #42264, #25589 ) ;
#51995=CARTESIAN_POINT ( 'NONE',  ( -26.00000000000000000, 0.000000000000000000, -2.818925648462311923E-15 ) ) ;
#52051=CARTESIAN_POINT ( 'NONE',  ( 0.000000000000000000, 0.000000000000000000, 0.000000000000000000 ) ) ;
#52161=ORIENTED_EDGE ( 'NONE', *, *, #17452, .T. ) ;
#52331=VECTOR ( 'NONE', #24499, 999.9999999999998863 ) ;
#52490=EDGE_LOOP ( 'NONE', ( #52507, #64571, #52161, #7029 ) ) ;
#52507=ORIENTED_EDGE ( 'NONE', *, *, #63069, .F. ) ;
#52603=SHAPE_DEFINITION_REPRESENTATION ( #3588, #48255 ) ;
#52700=CARTESIAN_POINT ( 'NONE',  ( -12.99999999999999822, 0.000000000000000000, -17.00000000000000355 ) ) ;
#52737=VERTEX_POINT ( 'NONE', #30876 ) ;
#52799=DIRECTION ( 'NONE',  ( 0.000000000000000000, -0.7660444431189770143, 0.6427876096865403621 ) ) ;
#52944=ORIENTED_EDGE ( 'NONE', *, *, #42506, .F. ) ;
#53071=PLANE ( 'NONE',  #29201 ) ;
#53129=VECTOR ( 'NONE', #33653, 1000.000000000000114 ) ;
#53148=DIRECTION ( 'NONE',  ( 0.000000000000000000, 0.000000000000000000, -1.000000000000000000 ) ) ;
#53164=LINE ( 'NONE', #30703, #49580 ) ;
#53300=LINE ( 'NONE', #59277, #67929 ) ;
#53368=DIRECTION ( 'NONE',  ( -1.000000000000000000, 0.000000000000000000, -2.168404344971009361E-16 ) ) ;
#53508=VERTEX_POINT ( 'NONE', #66727 ) ;
#53619=VECTOR ( 'NONE', #4213, 1000.000000000000000 ) ;
#53706=CARTESIAN_POINT ( 'NONE',  ( -25.99999999999999645, 1.117010584002392767E-15, -17.00000000000000355 ) ) ;
#53817=EDGE_CURVE ( 'NONE', #41104, #10412, #6752, .T. ) ;
#53975=AXIS2_PLACEMENT_3D ( 'NONE', #51007, #45376, #67533 ) ;
#54186=DIRECTION ( 'NONE',  ( -0.6427876096865403621, -0.7660444431189770143, 0.000000000000000000 ) ) ;
#54222=CARTESIAN_POINT ( 'NONE',  ( 39.99999999999997868, 29.79383981485517197, -1.218703225458906021E-14 ) ) ;
#54236=CARTESIAN_POINT ( 'NONE',  ( -26.00000000000002132, 0.000000000000000000, 55.00000000000001421 ) ) ;
#54242=VERTEX_POINT ( 'NONE', #45256 ) ;
#54454=DIRECTION ( 'NONE',  ( -0.7660444431189771253, 0.6427876096865404731, 0.000000000000000000 ) ) ;
#54456=ORIENTED_EDGE ( 'NONE', *, *, #32879, .T. ) ;
#54749=ORIENTED_EDGE ( 'NONE', *, *, #30834, .T. ) ;
#54818=SURFACE_STYLE_FILL_AREA ( #65392 ) ;
#54826=CARTESIAN_POINT ( 'NONE',  ( -40.99999999999999289, 0.000000000000000000, 55.00000000000001421 ) ) ;
#55245=CARTESIAN_POINT ( 'NONE',  ( -90.99999999999998579, 0.000000000000000000, -2.818925648462311528E-14 ) ) ;
#55696=ORIENTED_EDGE ( 'NONE', *, *, #16445, .F. ) ;
#55760=PRODUCT_DEFINITION_FORMATION_WITH_SPECIFIED_SOURCE ( 'ANY', '', #30563, .NOT_KNOWN. ) ;
#55764=VECTOR ( 'NONE', #69183, 1000.000000000000114 ) ;
#55768=LINE ( 'NONE', #1965, #39899 ) ;
#55788=DIRECTION ( 'NONE',  ( 0.000000000000000000, 0.000000000000000000, -1.000000000000000000 ) ) ;
#55901=( BOUNDED_CURVE ( )  B_SPLINE_CURVE ( 3, ( #27164, #64116, #22247, #11331 ),
 .UNSPECIFIED., .F., .F. ) 
 B_SPLINE_CURVE_WITH_KNOTS ( ( 4, 4 ),
 ( 2.398060303794313342, 2.801953471882904001 ),
 .UNSPECIFIED. ) 
 CURVE ( )  GEOMETRIC_REPRESENTATION_ITEM ( )  RATIONAL_B_SPLINE_CURVE ( ( 1.000000000000000000, 0.9864519964717846090, 0.9864519964717846090, 1.000000000000000000 ) ) 
 REPRESENTATION_ITEM ( '' )  );
#55915=EDGE_CURVE ( 'NONE', #37097, #7708, #1497, .T. ) ;
#56069=VERTEX_POINT ( 'NONE', #28104 ) ;
#56112=CARTESIAN_POINT ( 'NONE',  ( 39.99999999999999289, 29.79383981485516486, 30.00000000000001066 ) ) ;
#56127=VECTOR ( 'NONE', #64332, 1000.000000000000114 ) ;
#56352=AXIS2_PLACEMENT_3D ( 'NONE', #18712, #1484, #56688 ) ;
#56469=EDGE_CURVE ( 'NONE', #41104, #42670, #53300, .T. ) ;
#56636=CARTESIAN_POINT ( 'NONE',  ( -40.99999999999996447, 0.000000000000000000, -6.071532165918820097E-15 ) ) ;
#56688=DIRECTION ( 'NONE',  ( 0.000000000000000000, -0.000000000000000000, -1.000000000000000000 ) ) ;
#56742=ORIENTED_EDGE ( 'NONE', *, *, #14076, .T. ) ;
#56805=DIRECTION ( 'NONE',  ( 0.6427876096865403621, 0.7660444431189770143, 8.577375050694297349E-17 ) ) ;
#56913=VECTOR ( 'NONE', #56929, 1000.000000000000000 ) ;
#56929=DIRECTION ( 'NONE',  ( -0.5407162030609373726, -0.6444004775717706579, 0.5407162030609374836 ) ) ;
#56987=LINE ( 'NONE', #52051, #53619 ) ;
#57134=EDGE_LOOP ( 'NONE', ( #20242, #32666, #16321, #54749, #16017, #64596, #2191, #43024, #10439, #50409, #63331, #7927, #27459, #48777, #68553, #50564, #23322, #2230, #39645, #7077 ) ) ;
#57218=ORIENTED_EDGE ( 'NONE', *, *, #61959, .T. ) ;
#57319=CARTESIAN_POINT ( 'NONE',  ( -25.99999999999999289, 0.000000000000000000, -17.00000000000000711 ) ) ;
#57398=ORIENTED_EDGE ( 'NONE', *, *, #1761, .T. ) ;
#57416=CARTESIAN_POINT ( 'NONE',  ( 39.99999999999996447, 29.79383981485516486, -79.99999999999998579 ) ) ;
#57463=VECTOR ( 'NONE', #27596, 1000.000000000000000 ) ;
#57568=LINE ( 'NONE', #9378, #51054 ) ;
#57751=DIRECTION ( 'NONE',  ( 0.000000000000000000, 0.000000000000000000, 1.000000000000000000 ) ) ;
#58013=CARTESIAN_POINT ( 'NONE',  ( -40.99999999999996447, 0.000000000000000000, -6.071532165918820097E-15 ) ) ;
#58094=PLANE ( 'NONE',  #30311 ) ;
#58312=CARTESIAN_POINT ( 'NONE',  ( -26.00000000000000000, 0.000000000000000000, -2.818925648462311923E-15 ) ) ;
#58349=EDGE_LOOP ( 'NONE', ( #44822, #12293, #22651, #26772, #65025 ) ) ;
#58373=VECTOR ( 'NONE', #11826, 1000.000000000000000 ) ;
#58445=DIRECTION ( 'NONE',  ( -0.6427876096865403621, -0.7660444431189770143, 0.000000000000000000 ) ) ;
#58454=EDGE_CURVE ( 'NONE', #52737, #37939, #2144, .T. ) ;
#58459=EDGE_CURVE ( 'NONE', #19218, #26538, #40118, .T. ) ;
#58595=ORIENTED_EDGE ( 'NONE', *, *, #40986, .T. ) ;
#58664=CARTESIAN_POINT ( 'NONE',  ( 0.000000000000000000, 0.000000000000000000, 0.000000000000000000 ) ) ;
#58696=CARTESIAN_POINT ( 'NONE',  ( -40.99999999999997868, 0.000000000000000000, -6.071532165918823253E-15 ) ) ;
#58739=CARTESIAN_POINT ( 'NONE',  ( -63.76691715686636996, 29.79383981485516841, -25.00000000000000711 ) ) ;
#58963=CARTESIAN_POINT ( 'NONE',  ( -12.99999999999999645, 10.00000000000000000, -33.00000000000000000 ) ) ;
#59277=CARTESIAN_POINT ( 'NONE',  ( 39.99999999999999289, 29.79383981485516841, -5.248138350681833405E-15 ) ) ;
#59288=LINE ( 'NONE', #11437, #30919 ) ;
#59613=EDGE_CURVE ( 'NONE', #49963, #56069, #2515, .T. ) ;
#59688=DIRECTION ( 'NONE',  ( 0.000000000000000000, 0.000000000000000000, 1.000000000000000000 ) ) ;
#59820=FACE_OUTER_BOUND ( 'NONE', #4737, .T. ) ;
#60086=CARTESIAN_POINT ( 'NONE',  ( 10.61438981621043531, -5.226566692248933776, 4.385610183789550476 ) ) ;
#60153=EDGE_LOOP ( 'NONE', ( #47538, #22962, #27198, #16217, #67561 ) ) ;
#60246=CARTESIAN_POINT ( 'NONE',  ( 0.000000000000000000, 0.000000000000000000, 0.000000000000000000 ) ) ;
#60335=ADVANCED_FACE ( 'NONE', ( #48330 ), #21623, .T. ) ;
#60378=ORIENTED_EDGE ( 'NONE', *, *, #58459, .F. ) ;
#60604=FACE_OUTER_BOUND ( 'NONE', #10345, .T. ) ;
#60650=SHAPE_REPRESENTATION_RELATIONSHIP ( 'NONE' , 'NONE' ,  #48255, #50824 ) ;
#60955=VERTEX_POINT ( 'NONE', #43857 ) ;
#61177=VECTOR ( 'NONE', #37151, 1000.000000000000000 ) ;
#61247=EDGE_CURVE ( 'NONE', #10412, #27437, #44117, .T. ) ;
#61255=ORIENTED_EDGE ( 'NONE', *, *, #13823, .T. ) ;
#61406=CYLINDRICAL_SURFACE ( 'NONE', #39647, 75.00000000000001421 ) ;
#61559=EDGE_CURVE ( 'NONE', #56069, #14782, #11336, .T. ) ;
#61612=CARTESIAN_POINT ( 'NONE',  ( -90.99999999999994316, 0.000000000000000000, -105.0000000000000142 ) ) ;
#61855=EDGE_CURVE ( 'NONE', #42670, #4994, #9083, .T. ) ;
#61857=EDGE_CURVE ( 'NONE', #7708, #19981, #193, .T. ) ;
#61959=EDGE_CURVE ( 'NONE', #37939, #19637, #27104, .T. ) ;
#62209=ORIENTED_EDGE ( 'NONE', *, *, #59613, .T. ) ;
#62222=LINE ( 'NONE', #41124, #19348 ) ;
#62229=EDGE_CURVE ( 'NONE', #19637, #2392, #46225, .T. ) ;
#62478=EDGE_LOOP ( 'NONE', ( #12294, #64356, #62209 ) ) ;
#62534=VECTOR ( 'NONE', #48957, 1000.000000000000000 ) ;
#62592=DIRECTION ( 'NONE',  ( 0.000000000000000000, 0.000000000000000000, 1.000000000000000000 ) ) ;
#62716=CARTESIAN_POINT ( 'NONE',  ( 64.99999999999997158, 0.000000000000000000, -105.0000000000000000 ) ) ;
#62719=CARTESIAN_POINT ( 'NONE',  ( 21.57182537987927162, 17.67134260003770052, -14.82801705809902515 ) ) ;
#62728=EDGE_CURVE ( 'NONE', #62792, #16895, #19505, .T. ) ;
#62792=VERTEX_POINT ( 'NONE', #10324 ) ;
#62968=VERTEX_POINT ( 'NONE', #39160 ) ;
#63069=EDGE_CURVE ( 'NONE', #65127, #16895, #51781, .T. ) ;
#63331=ORIENTED_EDGE ( 'NONE', *, *, #28757, .F. ) ;
#63346=VECTOR ( 'NONE', #62592, 1000.000000000000000 ) ;
#63402=PLANE ( 'NONE',  #30720 ) ;
#63719=VECTOR ( 'NONE', #10830, 1000.000000000000000 ) ;
#63739=CARTESIAN_POINT ( 'NONE',  ( 14.99999999999998579, 0.000000000000000000, 0.000000000000000000 ) ) ;
#63872=AXIS2_PLACEMENT_3D ( 'NONE', #32800, #793, #37726 ) ;
#64070=DIRECTION ( 'NONE',  ( -1.000000000000000000, 0.000000000000000000, -0.000000000000000000 ) ) ;
#64116=CARTESIAN_POINT ( 'NONE',  ( -56.28348399776042044, 22.91216519805203333, -19.22558936715843814 ) ) ;
#64231=EDGE_LOOP ( 'NONE', ( #67264, #21859, #35810 ) ) ;
#64315=FACE_OUTER_BOUND ( 'NONE', #60153, .T. ) ;
#64332=DIRECTION ( 'NONE',  ( -0.5407162030609373726, -0.6444004775717707689, 0.5407162030609373726 ) ) ;
#64356=ORIENTED_EDGE ( 'NONE', *, *, #38290, .F. ) ;
#64540=DIRECTION ( 'NONE',  ( 1.000000000000000000, 0.000000000000000000, 1.334402673828313339E-16 ) ) ;
#64571=ORIENTED_EDGE ( 'NONE', *, *, #21371, .F. ) ;
#64596=ORIENTED_EDGE ( 'NONE', *, *, #61559, .F. ) ;
#64725=EDGE_CURVE ( 'NONE', #41104, #49158, #68457, .T. ) ;
#64829=ORIENTED_EDGE ( 'NONE', *, *, #63069, .T. ) ;
#64893=DIRECTION ( 'NONE',  ( -1.334402673828313339E-16, 0.000000000000000000, 1.000000000000000000 ) ) ;
#64953=DIRECTION ( 'NONE',  ( 1.000000000000000000, 0.000000000000000000, 0.000000000000000000 ) ) ;
#65000=LINE ( 'NONE', #58664, #63719 ) ;
#65025=ORIENTED_EDGE ( 'NONE', *, *, #6808, .F. ) ;
#65127=VERTEX_POINT ( 'NONE', #4687 ) ;
#65221=VERTEX_POINT ( 'NONE', #9978 ) ;
#65392=FILL_AREA_STYLE ('',( #6640 ) ) ;
#65533=ORIENTED_EDGE ( 'NONE', *, *, #46190, .T. ) ;
#65548=STYLED_ITEM ( 'NONE', ( #27741 ), #39903 ) ;
#65599=CARTESIAN_POINT ( 'NONE',  ( -25.99999999999994671, 0.000000000000000000, -104.9999999999999858 ) ) ;
#65618=EDGE_CURVE ( 'NONE', #2392, #26538, #11515, .T. ) ;
#65714=ORIENTED_EDGE ( 'NONE', *, *, #58454, .F. ) ;
#65747=( NAMED_UNIT ( * ) PLANE_ANGLE_UNIT ( ) SI_UNIT ( $, .RADIAN. ) );
#65828=DIRECTION ( 'NONE',  ( -3.903127820947816455E-16, 0.000000000000000000, 1.000000000000000000 ) ) ;
#66053=DIRECTION ( 'NONE',  ( 0.000000000000000000, 1.000000000000000000, -0.000000000000000000 ) ) ;
#66126=LINE ( 'NONE', #69374, #12724 ) ;
#66301=VECTOR ( 'NONE', #21762, 1000.000000000000000 ) ;
#66369=EDGE_CURVE ( 'NONE', #65221, #45932, #44413, .T. ) ;
#66568=FACE_OUTER_BOUND ( 'NONE', #52490, .T. ) ;
#66727=CARTESIAN_POINT ( 'NONE',  ( -40.99999999999997868, 0.000000000000000000, -6.071532165918823253E-15 ) ) ;
#66728=CARTESIAN_POINT ( 'NONE',  ( 39.99999999999997158, 29.79383981485516131, -25.00000000000000000 ) ) ;
#66752=VERTEX_POINT ( 'NONE', #57319 ) ;
#66765=VECTOR ( 'NONE', #25505, 1000.000000000000114 ) ;
#66785=ORIENTED_EDGE ( 'NONE', *, *, #42769, .T. ) ;
#66800=ADVANCED_FACE ( 'NONE', ( #46064 ), #8444, .F. ) ;
#66832=AXIS2_PLACEMENT_3D ( 'NONE', #50530, #44558, #8319 ) ;
#66916=PLANE ( 'NONE',  #56352 ) ;
#66933=DIRECTION ( 'NONE',  ( -0.5407162030609373726, -0.6444004775717707689, -0.5407162030609373726 ) ) ;
#66986=ADVANCED_FACE ( 'NONE', ( #64315 ), #26347, .T. ) ;
#67264=ORIENTED_EDGE ( 'NONE', *, *, #37541, .T. ) ;
#67405=DIRECTION ( 'NONE',  ( 0.7660444431189771253, 0.6427876096865404731, 1.661094098900087138E-16 ) ) ;
#67533=DIRECTION ( 'NONE',  ( -1.000000000000000000, 0.000000000000000000, 0.000000000000000000 ) ) ;
#67561=ORIENTED_EDGE ( 'NONE', *, *, #30027, .T. ) ;
#67929=VECTOR ( 'NONE', #4784, 1000.000000000000000 ) ;
#68042=ORIENTED_EDGE ( 'NONE', *, *, #61857, .F. ) ;
#68050=DIRECTION ( 'NONE',  ( 0.6427876096865403621, 0.7660444431189770143, 1.393823445737823288E-16 ) ) ;
#68126=DIRECTION ( 'NONE',  ( -0.5407162030609373726, -0.6444004775717707689, -0.5407162030609373726 ) ) ;
#68181=CARTESIAN_POINT ( 'NONE',  ( 31.08057067389502137, 19.16407787157944398, 38.91942932610497508 ) ) ;
#68228=DIRECTION ( 'NONE',  ( 0.000000000000000000, -0.7660444431189770143, 0.6427876096865403621 ) ) ;
#68457=LINE ( 'NONE', #40676, #47101 ) ;
#68553=ORIENTED_EDGE ( 'NONE', *, *, #44711, .F. ) ;
#68930=PLANE ( 'NONE',  #46469 ) ;
#68999=AXIS2_PLACEMENT_3D ( 'NONE', #47942, #69413, #68050 ) ;
#69183=DIRECTION ( 'NONE',  ( 0.5407162030609372616, -0.6444004775717707689, 0.5407162030609374836 ) ) ;
#69374=CARTESIAN_POINT ( 'NONE',  ( 0.000000000000000000, 0.000000000000000000, 0.000000000000000000 ) ) ;
#69413=DIRECTION ( 'NONE',  ( -0.7660444431189771253, 0.6427876096865404731, -2.989969378020156799E-16 ) ) ;
ENDSEC;
END-ISO-10303-21;
